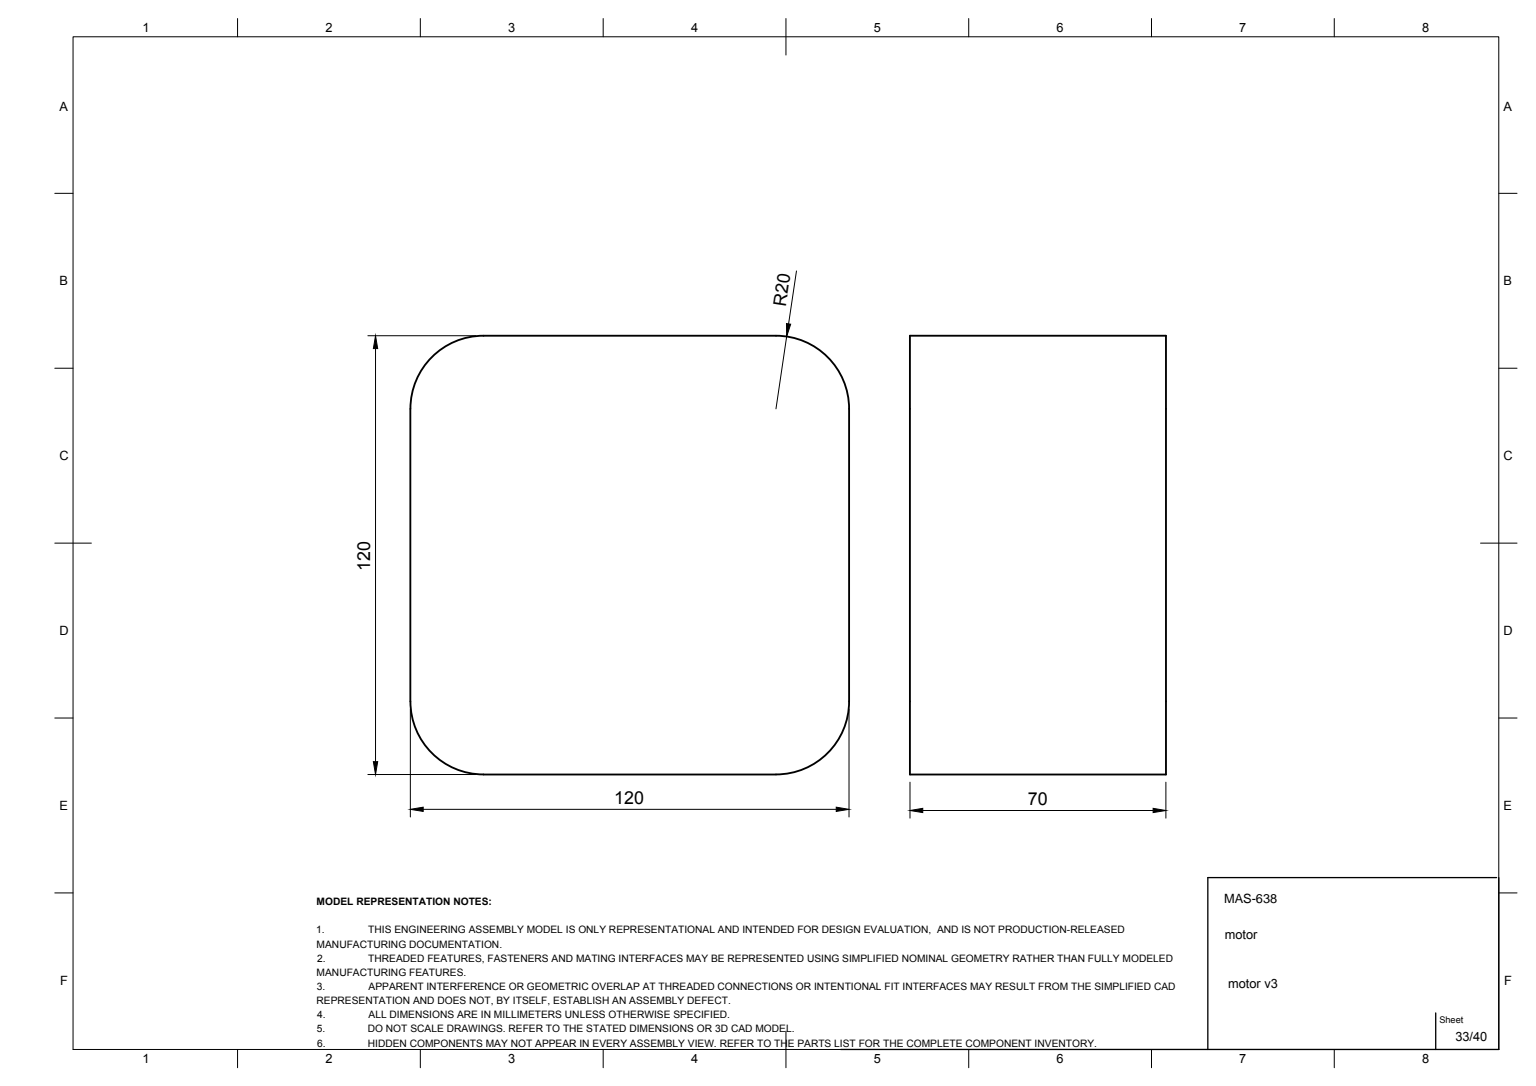
ISO-10303-21;
HEADER;
FILE_DESCRIPTION((''),'2;1');
FILE_NAME('Motor.step','2026-10-09T12:00:21-07:00',(''),(''),'','','');
FILE_SCHEMA (('AUTOMOTIVE_DESIGN { 1 0 10303 214 3 1 1 }'));
ENDSEC;
DATA;
#10=MECHANICAL_DESIGN_GEOMETRIC_PRESENTATION_REPRESENTATION('',(#430),#10334);
#147=CYLINDRICAL_SURFACE('',#4162,2.) ;
#148=CYLINDRICAL_SURFACE('',#4163,2.) ;
#149=CYLINDRICAL_SURFACE('',#4164,2.) ;
#150=CYLINDRICAL_SURFACE('',#4165,2.) ;
#358=SHAPE_REPRESENTATION_RELATIONSHIP('SRR','None',#10475,#390) ;
#390=ADVANCED_BREP_SHAPE_REPRESENTATION('',(#462),#10327) ;
#430=STYLED_ITEM('',(#10631),#462) ;
#462=MANIFOLD_SOLID_BREP('Body1',#3584) ;
#492=PLANE('',#4148) ;
#493=PLANE('',#4149) ;
#494=PLANE('',#4150) ;
#495=PLANE('',#4151) ;
#496=PLANE('',#4152) ;
#497=PLANE('',#4157) ;
#569=LINE('',#9677,#727) ;
#570=LINE('',#9679,#728) ;
#571=LINE('',#9681,#729) ;
#572=LINE('',#9682,#730) ;
#573=LINE('',#9686,#731) ;
#574=LINE('',#9688,#732) ;
#575=LINE('',#9690,#733) ;
#576=LINE('',#9691,#734) ;
#577=LINE('',#9695,#735) ;
#578=LINE('',#9697,#736) ;
#579=LINE('',#9699,#737) ;
#580=LINE('',#9700,#738) ;
#581=LINE('',#9704,#739) ;
#582=LINE('',#9706,#740) ;
#583=LINE('',#9708,#741) ;
#584=LINE('',#9709,#742) ;
#727=VECTOR('',#4893,100.) ;
#728=VECTOR('',#4894,100.) ;
#729=VECTOR('',#4895,100.) ;
#730=VECTOR('',#4896,100.) ;
#731=VECTOR('',#4899,100.) ;
#732=VECTOR('',#4900,100.) ;
#733=VECTOR('',#4901,100.) ;
#734=VECTOR('',#4902,100.) ;
#735=VECTOR('',#4905,100.) ;
#736=VECTOR('',#4906,100.) ;
#737=VECTOR('',#4907,100.) ;
#738=VECTOR('',#4908,100.) ;
#739=VECTOR('',#4911,100.) ;
#740=VECTOR('',#4912,100.) ;
#741=VECTOR('',#4913,100.) ;
#742=VECTOR('',#4914,100.) ;
#933=FACE_OUTER_BOUND('',#1139,.T.) ;
#934=FACE_OUTER_BOUND('',#1140,.T.) ;
#935=FACE_OUTER_BOUND('',#1141,.T.) ;
#936=FACE_OUTER_BOUND('',#1142,.T.) ;
#937=FACE_OUTER_BOUND('',#1143,.T.) ;
#938=FACE_OUTER_BOUND('',#1144,.T.) ;
#939=FACE_OUTER_BOUND('',#1145,.T.) ;
#940=FACE_OUTER_BOUND('',#1146,.T.) ;
#941=FACE_OUTER_BOUND('',#1147,.T.) ;
#942=FACE_OUTER_BOUND('',#1148,.T.) ;
#1139=EDGE_LOOP('',(#2735,#2736,#2737,#2738)) ;
#1140=EDGE_LOOP('',(#2739,#2740,#2741,#2742)) ;
#1141=EDGE_LOOP('',(#2743,#2744,#2745,#2746)) ;
#1142=EDGE_LOOP('',(#2747,#2748,#2749,#2750)) ;
#1143=EDGE_LOOP('',(#2751,#2752,#2753,#2754,#2755,#2756,#2757,#2758)) ;
#1144=EDGE_LOOP('',(#2759,#2760,#2761,#2762,#2763,#2764,#2765,#2766)) ;
#1145=EDGE_LOOP('',(#2767,#2768,#2769,#2770)) ;
#1146=EDGE_LOOP('',(#2771,#2772,#2773,#2774)) ;
#1147=EDGE_LOOP('',(#2775,#2776,#2777,#2778)) ;
#1148=EDGE_LOOP('',(#2779,#2780,#2781,#2782)) ;
#1337=CIRCLE('',#4153,2.) ;
#1338=CIRCLE('',#4154,2.) ;
#1339=CIRCLE('',#4155,2.) ;
#1340=CIRCLE('',#4156,2.) ;
#1341=CIRCLE('',#4158,2.) ;
#1342=CIRCLE('',#4159,2.) ;
#1343=CIRCLE('',#4160,2.) ;
#1344=CIRCLE('',#4161,2.) ;
#1640=VERTEX_POINT('',#9675) ;
#1641=VERTEX_POINT('',#9676) ;
#1642=VERTEX_POINT('',#9678) ;
#1643=VERTEX_POINT('',#9680) ;
#1644=VERTEX_POINT('',#9684) ;
#1645=VERTEX_POINT('',#9685) ;
#1646=VERTEX_POINT('',#9687) ;
#1647=VERTEX_POINT('',#9689) ;
#1648=VERTEX_POINT('',#9693) ;
#1649=VERTEX_POINT('',#9694) ;
#1650=VERTEX_POINT('',#9696) ;
#1651=VERTEX_POINT('',#9698) ;
#1652=VERTEX_POINT('',#9702) ;
#1653=VERTEX_POINT('',#9703) ;
#1654=VERTEX_POINT('',#9705) ;
#1655=VERTEX_POINT('',#9707) ;
#2024=EDGE_CURVE('',#1640,#1641,#569,.T.) ;
#2025=EDGE_CURVE('',#1641,#1642,#570,.T.) ;
#2026=EDGE_CURVE('',#1643,#1642,#571,.T.) ;
#2027=EDGE_CURVE('',#1643,#1640,#572,.T.) ;
#2028=EDGE_CURVE('',#1644,#1645,#573,.T.) ;
#2029=EDGE_CURVE('',#1645,#1646,#574,.T.) ;
#2030=EDGE_CURVE('',#1647,#1646,#575,.T.) ;
#2031=EDGE_CURVE('',#1647,#1644,#576,.T.) ;
#2032=EDGE_CURVE('',#1648,#1649,#577,.T.) ;
#2033=EDGE_CURVE('',#1648,#1650,#578,.T.) ;
#2034=EDGE_CURVE('',#1650,#1651,#579,.T.) ;
#2035=EDGE_CURVE('',#1651,#1649,#580,.T.) ;
#2036=EDGE_CURVE('',#1652,#1653,#581,.T.) ;
#2037=EDGE_CURVE('',#1653,#1654,#582,.T.) ;
#2038=EDGE_CURVE('',#1655,#1654,#583,.T.) ;
#2039=EDGE_CURVE('',#1655,#1652,#584,.T.) ;
#2040=EDGE_CURVE('',#1646,#1648,#1337,.T.) ;
#2041=EDGE_CURVE('',#1649,#1655,#1338,.T.) ;
#2042=EDGE_CURVE('',#1654,#1643,#1339,.T.) ;
#2043=EDGE_CURVE('',#1642,#1647,#1340,.T.) ;
#2044=EDGE_CURVE('',#1650,#1645,#1341,.T.) ;
#2045=EDGE_CURVE('',#1644,#1641,#1342,.T.) ;
#2046=EDGE_CURVE('',#1640,#1653,#1343,.T.) ;
#2047=EDGE_CURVE('',#1652,#1651,#1344,.T.) ;
#2735=ORIENTED_EDGE('',*,*,#2024,.T.) ;
#2736=ORIENTED_EDGE('',*,*,#2025,.T.) ;
#2737=ORIENTED_EDGE('',*,*,#2026,.F.) ;
#2738=ORIENTED_EDGE('',*,*,#2027,.T.) ;
#2739=ORIENTED_EDGE('',*,*,#2028,.T.) ;
#2740=ORIENTED_EDGE('',*,*,#2029,.T.) ;
#2741=ORIENTED_EDGE('',*,*,#2030,.F.) ;
#2742=ORIENTED_EDGE('',*,*,#2031,.T.) ;
#2743=ORIENTED_EDGE('',*,*,#2032,.F.) ;
#2744=ORIENTED_EDGE('',*,*,#2033,.T.) ;
#2745=ORIENTED_EDGE('',*,*,#2034,.T.) ;
#2746=ORIENTED_EDGE('',*,*,#2035,.T.) ;
#2747=ORIENTED_EDGE('',*,*,#2036,.T.) ;
#2748=ORIENTED_EDGE('',*,*,#2037,.T.) ;
#2749=ORIENTED_EDGE('',*,*,#2038,.F.) ;
#2750=ORIENTED_EDGE('',*,*,#2039,.T.) ;
#2751=ORIENTED_EDGE('',*,*,#2030,.T.) ;
#2752=ORIENTED_EDGE('',*,*,#2040,.T.) ;
#2753=ORIENTED_EDGE('',*,*,#2032,.T.) ;
#2754=ORIENTED_EDGE('',*,*,#2041,.T.) ;
#2755=ORIENTED_EDGE('',*,*,#2038,.T.) ;
#2756=ORIENTED_EDGE('',*,*,#2042,.T.) ;
#2757=ORIENTED_EDGE('',*,*,#2026,.T.) ;
#2758=ORIENTED_EDGE('',*,*,#2043,.T.) ;
#2759=ORIENTED_EDGE('',*,*,#2034,.F.) ;
#2760=ORIENTED_EDGE('',*,*,#2044,.T.) ;
#2761=ORIENTED_EDGE('',*,*,#2028,.F.) ;
#2762=ORIENTED_EDGE('',*,*,#2045,.T.) ;
#2763=ORIENTED_EDGE('',*,*,#2024,.F.) ;
#2764=ORIENTED_EDGE('',*,*,#2046,.T.) ;
#2765=ORIENTED_EDGE('',*,*,#2036,.F.) ;
#2766=ORIENTED_EDGE('',*,*,#2047,.T.) ;
#2767=ORIENTED_EDGE('',*,*,#2040,.F.) ;
#2768=ORIENTED_EDGE('',*,*,#2029,.F.) ;
#2769=ORIENTED_EDGE('',*,*,#2044,.F.) ;
#2770=ORIENTED_EDGE('',*,*,#2033,.F.) ;
#2771=ORIENTED_EDGE('',*,*,#2043,.F.) ;
#2772=ORIENTED_EDGE('',*,*,#2025,.F.) ;
#2773=ORIENTED_EDGE('',*,*,#2045,.F.) ;
#2774=ORIENTED_EDGE('',*,*,#2031,.F.) ;
#2775=ORIENTED_EDGE('',*,*,#2042,.F.) ;
#2776=ORIENTED_EDGE('',*,*,#2037,.F.) ;
#2777=ORIENTED_EDGE('',*,*,#2046,.F.) ;
#2778=ORIENTED_EDGE('',*,*,#2027,.F.) ;
#2779=ORIENTED_EDGE('',*,*,#2041,.F.) ;
#2780=ORIENTED_EDGE('',*,*,#2035,.F.) ;
#2781=ORIENTED_EDGE('',*,*,#2047,.F.) ;
#2782=ORIENTED_EDGE('',*,*,#2039,.F.) ;
#3441=ADVANCED_FACE('',(#933),#492,.F.) ;
#3442=ADVANCED_FACE('',(#934),#493,.F.) ;
#3443=ADVANCED_FACE('',(#935),#494,.F.) ;
#3444=ADVANCED_FACE('',(#936),#495,.F.) ;
#3445=ADVANCED_FACE('',(#937),#496,.T.) ;
#3446=ADVANCED_FACE('',(#938),#497,.F.) ;
#3447=ADVANCED_FACE('',(#939),#147,.T.) ;
#3448=ADVANCED_FACE('',(#940),#148,.T.) ;
#3449=ADVANCED_FACE('',(#941),#149,.T.) ;
#3450=ADVANCED_FACE('',(#942),#150,.T.) ;
#3584=CLOSED_SHELL('',(#3441,#3442,#3443,#3444,#3445,#3446,#3447,#3448,
#3449,#3450)) ;
#4147=AXIS2_PLACEMENT_3D('',#9673,#4889,#4890) ;
#4148=AXIS2_PLACEMENT_3D('',#9674,#4891,#4892) ;
#4149=AXIS2_PLACEMENT_3D('',#9683,#4897,#4898) ;
#4150=AXIS2_PLACEMENT_3D('',#9692,#4903,#4904) ;
#4151=AXIS2_PLACEMENT_3D('',#9701,#4909,#4910) ;
#4152=AXIS2_PLACEMENT_3D('',#9710,#4915,#4916) ;
#4153=AXIS2_PLACEMENT_3D('',#9711,#4917,#4918) ;
#4154=AXIS2_PLACEMENT_3D('',#9712,#4919,#4920) ;
#4155=AXIS2_PLACEMENT_3D('',#9713,#4921,#4922) ;
#4156=AXIS2_PLACEMENT_3D('',#9714,#4923,#4924) ;
#4157=AXIS2_PLACEMENT_3D('',#9715,#4925,#4926) ;
#4158=AXIS2_PLACEMENT_3D('',#9716,#4927,#4928) ;
#4159=AXIS2_PLACEMENT_3D('',#9717,#4929,#4930) ;
#4160=AXIS2_PLACEMENT_3D('',#9718,#4931,#4932) ;
#4161=AXIS2_PLACEMENT_3D('',#9719,#4933,#4934) ;
#4162=AXIS2_PLACEMENT_3D('',#9720,#4935,#4936) ;
#4163=AXIS2_PLACEMENT_3D('',#9721,#4937,#4938) ;
#4164=AXIS2_PLACEMENT_3D('',#9722,#4939,#4940) ;
#4165=AXIS2_PLACEMENT_3D('',#9723,#4941,#4942) ;
#4889=DIRECTION('axis',(0.,0.,1.)) ;
#4890=DIRECTION('refdir',(1.,0.,0.)) ;
#4891=DIRECTION('center_axis',(1.,4.03783642961741E-31,-1.15648231731787E-16)) ;
#4892=DIRECTION('ref_axis',(1.15648231731787E-16,-3.49148133884313E-15,
1.)) ;
#4893=DIRECTION('',(-1.15648231731787E-16,3.49148133884313E-15,-1.)) ;
#4894=DIRECTION('',(0.,-1.,-3.49148133884313E-15)) ;
#4895=DIRECTION('',(-1.15648231731787E-16,3.49148133884313E-15,-1.)) ;
#4896=DIRECTION('',(0.,1.,3.49148133884313E-15)) ;
#4897=DIRECTION('center_axis',(-1.73472347597681E-16,-3.49148133884313E-15,
1.)) ;
#4898=DIRECTION('ref_axis',(-1.,6.05675464442612E-31,-1.73472347597681E-16)) ;
#4899=DIRECTION('',(1.,-6.05675464442612E-31,1.73472347597681E-16)) ;
#4900=DIRECTION('',(0.,-1.,-3.49148133884313E-15)) ;
#4901=DIRECTION('',(1.,-6.05675464442612E-31,1.73472347597681E-16)) ;
#4902=DIRECTION('',(0.,1.,3.49148133884313E-15)) ;
#4903=DIRECTION('center_axis',(-1.,0.,0.)) ;
#4904=DIRECTION('ref_axis',(0.,-1.,-3.49148133884313E-15)) ;
#4905=DIRECTION('',(0.,-3.49148133884313E-15,1.)) ;
#4906=DIRECTION('',(0.,1.,3.49148133884313E-15)) ;
#4907=DIRECTION('',(0.,-3.49148133884313E-15,1.)) ;
#4908=DIRECTION('',(0.,-1.,-3.49148133884313E-15)) ;
#4909=DIRECTION('center_axis',(1.15648231731787E-16,3.49148133884313E-15,
-1.)) ;
#4910=DIRECTION('ref_axis',(1.,-4.03783642961741E-31,1.15648231731787E-16)) ;
#4911=DIRECTION('',(-1.,4.03783642961741E-31,-1.15648231731787E-16)) ;
#4912=DIRECTION('',(0.,-1.,-3.49148133884313E-15)) ;
#4913=DIRECTION('',(-1.,4.03783642961741E-31,-1.15648231731787E-16)) ;
#4914=DIRECTION('',(0.,1.,3.49148133884313E-15)) ;
#4915=DIRECTION('center_axis',(0.,-1.,-3.49148133884313E-15)) ;
#4916=DIRECTION('ref_axis',(1.,0.,0.)) ;
#4917=DIRECTION('center_axis',(0.,-1.,-3.49148133884313E-15)) ;
#4918=DIRECTION('ref_axis',(1.,0.,0.)) ;
#4919=DIRECTION('center_axis',(0.,-1.,-3.49148133884313E-15)) ;
#4920=DIRECTION('ref_axis',(1.,0.,0.)) ;
#4921=DIRECTION('center_axis',(0.,-1.,-3.49148133884313E-15)) ;
#4922=DIRECTION('ref_axis',(1.,0.,0.)) ;
#4923=DIRECTION('center_axis',(0.,-1.,-3.49148133884313E-15)) ;
#4924=DIRECTION('ref_axis',(1.,0.,0.)) ;
#4925=DIRECTION('center_axis',(0.,-1.,-3.49148133884313E-15)) ;
#4926=DIRECTION('ref_axis',(1.,0.,0.)) ;
#4927=DIRECTION('center_axis',(0.,1.,3.49148133884313E-15)) ;
#4928=DIRECTION('ref_axis',(1.,0.,0.)) ;
#4929=DIRECTION('center_axis',(0.,1.,3.49148133884313E-15)) ;
#4930=DIRECTION('ref_axis',(1.,0.,0.)) ;
#4931=DIRECTION('center_axis',(0.,1.,3.49148133884313E-15)) ;
#4932=DIRECTION('ref_axis',(1.,0.,0.)) ;
#4933=DIRECTION('center_axis',(0.,1.,3.49148133884313E-15)) ;
#4934=DIRECTION('ref_axis',(1.,0.,0.)) ;
#4935=DIRECTION('center_axis',(0.,1.,3.49148133884313E-15)) ;
#4936=DIRECTION('ref_axis',(-1.,0.,0.)) ;
#4937=DIRECTION('center_axis',(0.,1.,3.49148133884313E-15)) ;
#4938=DIRECTION('ref_axis',(-1.,0.,0.)) ;
#4939=DIRECTION('center_axis',(0.,1.,3.49148133884313E-15)) ;
#4940=DIRECTION('ref_axis',(-1.,0.,0.)) ;
#4941=DIRECTION('center_axis',(0.,1.,3.49148133884313E-15)) ;
#4942=DIRECTION('ref_axis',(-1.,0.,0.)) ;
#9673=CARTESIAN_POINT('',(0.,0.,0.)) ;
#9674=CARTESIAN_POINT('Origin',(17.47768801576,59.8830586252739,62.222433740001)) ;
#9675=CARTESIAN_POINT('',(17.47768801576,66.8830586252738,72.2224337400011)) ;
#9676=CARTESIAN_POINT('',(17.47768801576,66.8830586252739,64.2224337400011)) ;
#9677=CARTESIAN_POINT('',(17.47768801576,66.8830586252739,62.2224337400011)) ;
#9678=CARTESIAN_POINT('',(17.47768801576,59.8830586252739,64.2224337400011)) ;
#9679=CARTESIAN_POINT('',(17.47768801576,59.8830586252739,64.2224337400011)) ;
#9680=CARTESIAN_POINT('',(17.47768801576,59.8830586252738,72.222433740001)) ;
#9681=CARTESIAN_POINT('',(17.47768801576,59.8830586252739,62.222433740001)) ;
#9682=CARTESIAN_POINT('',(17.47768801576,59.8830586252738,72.222433740001)) ;
#9683=CARTESIAN_POINT('Origin',(29.47768801576,59.8830586252739,62.222433740001)) ;
#9684=CARTESIAN_POINT('',(19.47768801576,66.8830586252739,62.2224337400011)) ;
#9685=CARTESIAN_POINT('',(27.47768801576,66.8830586252739,62.2224337400011)) ;
#9686=CARTESIAN_POINT('',(29.47768801576,66.8830586252739,62.2224337400011)) ;
#9687=CARTESIAN_POINT('',(27.47768801576,59.8830586252739,62.222433740001)) ;
#9688=CARTESIAN_POINT('',(27.4776880157599,59.8830586252739,62.222433740001)) ;
#9689=CARTESIAN_POINT('',(19.47768801576,59.8830586252739,62.222433740001)) ;
#9690=CARTESIAN_POINT('',(29.47768801576,59.8830586252739,62.222433740001)) ;
#9691=CARTESIAN_POINT('',(19.47768801576,59.8830586252739,62.222433740001)) ;
#9692=CARTESIAN_POINT('Origin',(29.47768801576,59.8830586252739,62.222433740001)) ;
#9693=CARTESIAN_POINT('',(29.47768801576,59.8830586252739,64.2224337400011)) ;
#9694=CARTESIAN_POINT('',(29.47768801576,59.8830586252738,72.2224337400011)) ;
#9695=CARTESIAN_POINT('',(29.47768801576,59.8830586252739,62.222433740001)) ;
#9696=CARTESIAN_POINT('',(29.47768801576,66.8830586252739,64.2224337400011)) ;
#9697=CARTESIAN_POINT('',(29.47768801576,59.8830586252739,64.2224337400011)) ;
#9698=CARTESIAN_POINT('',(29.47768801576,66.8830586252738,72.2224337400011)) ;
#9699=CARTESIAN_POINT('',(29.47768801576,66.8830586252739,62.2224337400011)) ;
#9700=CARTESIAN_POINT('',(29.47768801576,59.8830586252738,72.2224337400011)) ;
#9701=CARTESIAN_POINT('Origin',(29.47768801576,59.8830586252738,74.2224337400011)) ;
#9702=CARTESIAN_POINT('',(27.4776880157599,66.8830586252738,74.2224337400011)) ;
#9703=CARTESIAN_POINT('',(19.47768801576,66.8830586252738,74.2224337400011)) ;
#9704=CARTESIAN_POINT('',(29.47768801576,66.8830586252738,74.2224337400011)) ;
#9705=CARTESIAN_POINT('',(19.47768801576,59.8830586252738,74.2224337400011)) ;
#9706=CARTESIAN_POINT('',(19.47768801576,59.8830586252738,74.2224337400011)) ;
#9707=CARTESIAN_POINT('',(27.4776880157599,59.8830586252738,74.2224337400011)) ;
#9708=CARTESIAN_POINT('',(29.47768801576,59.8830586252738,74.2224337400011)) ;
#9709=CARTESIAN_POINT('',(27.4776880157599,59.8830586252738,74.2224337400011)) ;
#9710=CARTESIAN_POINT('Origin',(23.47768801576,59.8830586252739,68.2224337400011)) ;
#9711=CARTESIAN_POINT('Origin',(27.4776880157599,59.8830586252739,64.2224337400011)) ;
#9712=CARTESIAN_POINT('Origin',(27.4776880157599,59.8830586252738,72.222433740001)) ;
#9713=CARTESIAN_POINT('Origin',(19.47768801576,59.8830586252738,72.222433740001)) ;
#9714=CARTESIAN_POINT('Origin',(19.47768801576,59.8830586252739,64.2224337400011)) ;
#9715=CARTESIAN_POINT('Origin',(23.47768801576,66.8830586252739,68.2224337400011)) ;
#9716=CARTESIAN_POINT('Origin',(27.4776880157599,66.8830586252739,64.2224337400011)) ;
#9717=CARTESIAN_POINT('Origin',(19.47768801576,66.8830586252739,64.2224337400011)) ;
#9718=CARTESIAN_POINT('Origin',(19.47768801576,66.8830586252738,72.2224337400011)) ;
#9719=CARTESIAN_POINT('Origin',(27.4776880157599,66.8830586252738,72.2224337400011)) ;
#9720=CARTESIAN_POINT('Origin',(27.4776880157599,59.8830586252739,64.2224337400011)) ;
#9721=CARTESIAN_POINT('Origin',(19.47768801576,59.8830586252739,64.2224337400011)) ;
#9722=CARTESIAN_POINT('Origin',(19.47768801576,59.8830586252738,72.222433740001)) ;
#9723=CARTESIAN_POINT('Origin',(27.4776880157599,59.8830586252738,72.222433740001)) ;
#10290=UNCERTAINTY_MEASURE_WITH_UNIT(LENGTH_MEASURE(0.001),#10335,
'DISTANCE_ACCURACY_VALUE',
'Maximum model space distance between geometric entities at asserted c
onnectivities') ;
#10297=UNCERTAINTY_MEASURE_WITH_UNIT(LENGTH_MEASURE(0.001),#10335,
'DISTANCE_ACCURACY_VALUE',
'Maximum model space distance between geometric entities at asserted c
onnectivities') ;
#10327=(
GEOMETRIC_REPRESENTATION_CONTEXT(3)
GLOBAL_UNCERTAINTY_ASSIGNED_CONTEXT((#10290))
GLOBAL_UNIT_ASSIGNED_CONTEXT((#10335,#10337,#10338))
REPRESENTATION_CONTEXT('','3D')
) ;
#10334=(
GEOMETRIC_REPRESENTATION_CONTEXT(3)
GLOBAL_UNCERTAINTY_ASSIGNED_CONTEXT((#10297))
GLOBAL_UNIT_ASSIGNED_CONTEXT((#10335,#10337,#10338))
REPRESENTATION_CONTEXT('','3D')
) ;
#10335=(
LENGTH_UNIT()
NAMED_UNIT(*)
SI_UNIT(.CENTI.,.METRE.)
) ;
#10337=(
NAMED_UNIT(*)
PLANE_ANGLE_UNIT()
SI_UNIT($,.RADIAN.)
) ;
#10338=(
NAMED_UNIT(*)
SI_UNIT($,.STERADIAN.)
SOLID_ANGLE_UNIT()
) ;
#10368=SHAPE_DEFINITION_REPRESENTATION(#10428,#10475) ;
#10428=PRODUCT_DEFINITION_SHAPE('',$,#10512) ;
#10475=SHAPE_REPRESENTATION('',(#4147),#10327) ;
#10482=PRODUCT_DEFINITION_CONTEXT('part definition',#10592,'design') ;
#10512=PRODUCT_DEFINITION('Motor','Motor',#10548,#10482) ;
#10548=PRODUCT_DEFINITION_FORMATION('',$,#10623) ;
#10592=APPLICATION_CONTEXT(
'Core Data for Automotive Mechanical Design Process') ;
#10593=PRODUCT_CONTEXT('part definition',#10592,'mechanical') ;
#10623=PRODUCT('Motor','Motor',$,(#10593)) ;
#10631=PRESENTATION_STYLE_ASSIGNMENT((#10635)) ;
#10635=SURFACE_STYLE_USAGE(.BOTH.,#10639) ;
#10639=SURFACE_SIDE_STYLE('',(#10643)) ;
#10643=SURFACE_STYLE_FILL_AREA(#10647) ;
#10647=FILL_AREA_STYLE('Opaque(25,25,25)',(#10651)) ;
#10651=FILL_AREA_STYLE_COLOUR('Opaque(25,25,25)',#10655) ;
#10655=COLOUR_RGB('Opaque(25,25,25)', 0.09019608, 0.27058824, 0.51372549) ;
ENDSEC;
END-ISO-10303-21;
